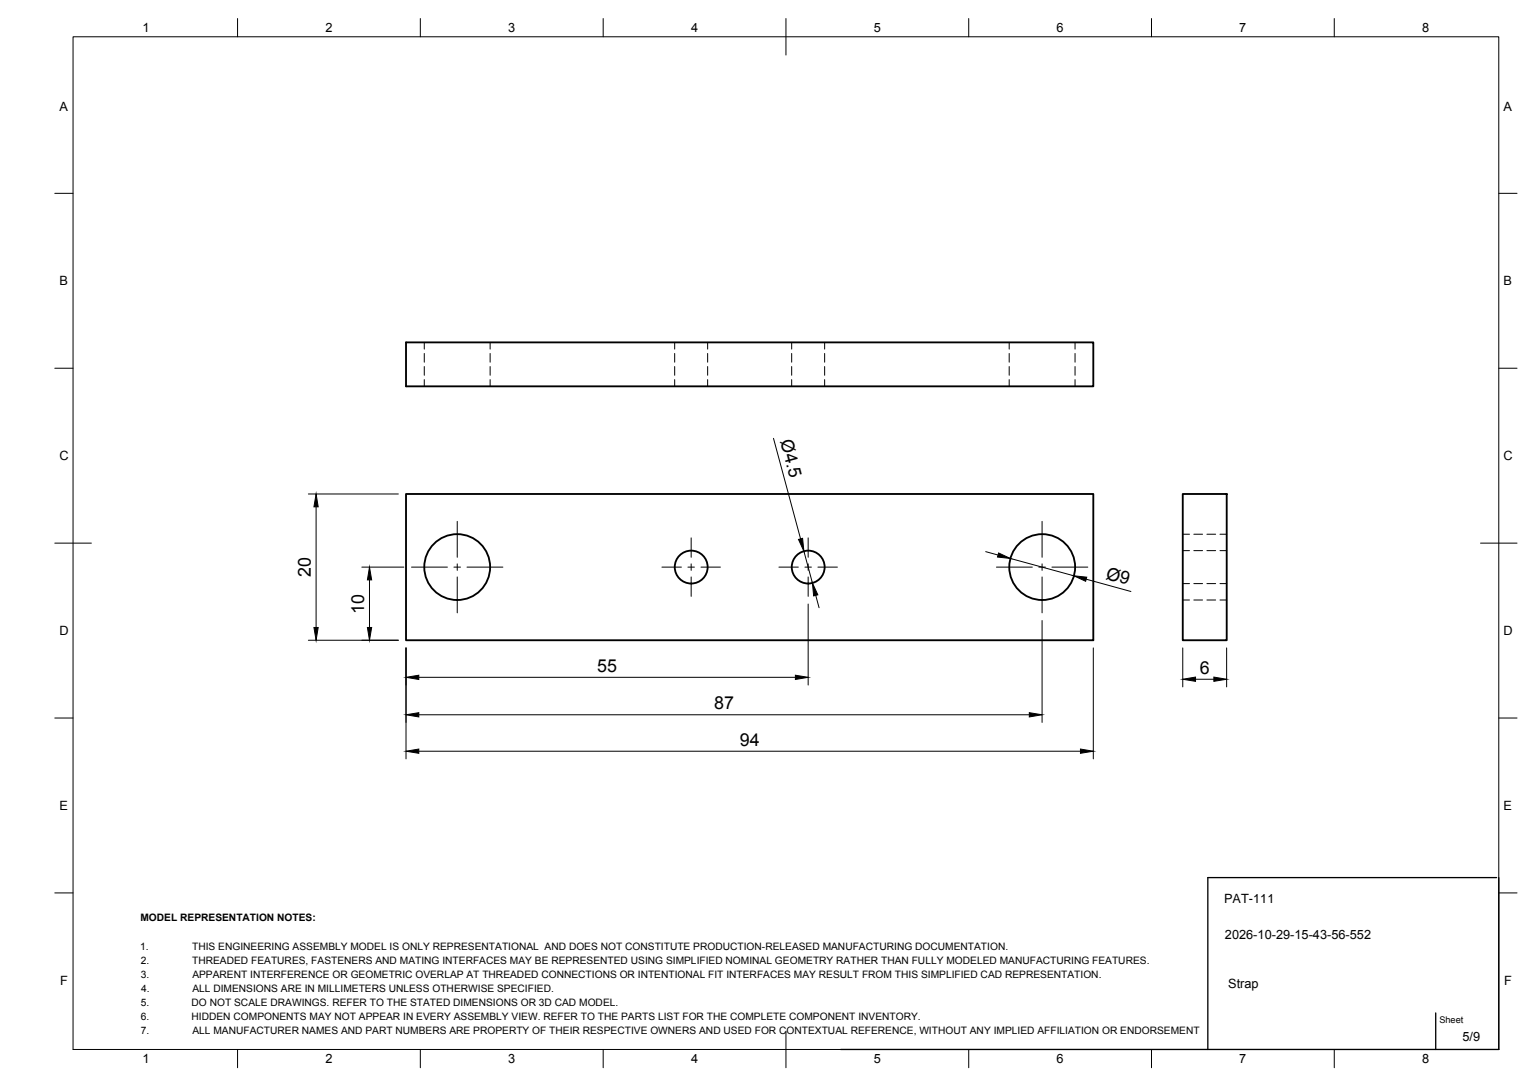
ISO-10303-21;
HEADER;
/* Generated by software containing ST-Developer
 * from STEP Tools, Inc. (www.steptools.com) 
 */

FILE_DESCRIPTION(
/* description */ ('Grid plate located blocks and clamp'),
/* implementation_level */ '2;1');

FILE_NAME(
/* name */ 'Strap.step',
/* time_stamp */ '2026-10-29T15:43:47-07:00',
/* author */ (''),
/* organization */ (''),
/* preprocessor_version */ 'ST-DEVELOPER v20.2',
/* originating_system */ 'Autodesk Translation Framework v15.17.0.0',
/* authorisation */ '');

FILE_SCHEMA (('AUTOMOTIVE_DESIGN { 1 0 10303 214 3 1 1 }'));
ENDSEC;

DATA;
#10=MECHANICAL_DESIGN_GEOMETRIC_PRESENTATION_REPRESENTATION('',(#172),#5702);
#146=SHAPE_REPRESENTATION_RELATIONSHIP('SRR','None',#5764,#158);
#158=ADVANCED_BREP_SHAPE_REPRESENTATION('',(#185),#5694);
#172=STYLED_ITEM('',(#5911),#185);
#185=MANIFOLD_SOLID_BREP('Body1',#3268);
#250=FACE_BOUND('',#811,.T.);
#251=FACE_BOUND('',#812,.T.);
#252=FACE_BOUND('',#813,.T.);
#253=FACE_BOUND('',#814,.T.);
#254=FACE_BOUND('',#816,.T.);
#255=FACE_BOUND('',#817,.T.);
#256=FACE_BOUND('',#818,.T.);
#257=FACE_BOUND('',#819,.T.);
#338=CIRCLE('',#3593,0.225);
#339=CIRCLE('',#3594,0.225);
#340=CIRCLE('',#3596,0.225);
#341=CIRCLE('',#3597,0.225);
#342=CIRCLE('',#3599,0.449999999999999);
#343=CIRCLE('',#3600,0.449999999999999);
#344=CIRCLE('',#3602,0.449999999999999);
#345=CIRCLE('',#3603,0.449999999999999);
#430=CYLINDRICAL_SURFACE('',#3592,0.225);
#431=CYLINDRICAL_SURFACE('',#3595,0.225);
#432=CYLINDRICAL_SURFACE('',#3598,0.449999999999999);
#433=CYLINDRICAL_SURFACE('',#3601,0.449999999999999);
#561=FACE_OUTER_BOUND('',#802,.T.);
#562=FACE_OUTER_BOUND('',#803,.T.);
#563=FACE_OUTER_BOUND('',#804,.T.);
#564=FACE_OUTER_BOUND('',#805,.T.);
#565=FACE_OUTER_BOUND('',#806,.T.);
#566=FACE_OUTER_BOUND('',#807,.T.);
#567=FACE_OUTER_BOUND('',#808,.T.);
#568=FACE_OUTER_BOUND('',#809,.T.);
#569=FACE_OUTER_BOUND('',#810,.T.);
#570=FACE_OUTER_BOUND('',#815,.T.);
#802=EDGE_LOOP('',(#2632,#2633,#2634,#2635));
#803=EDGE_LOOP('',(#2636,#2637,#2638,#2639));
#804=EDGE_LOOP('',(#2640,#2641,#2642,#2643));
#805=EDGE_LOOP('',(#2644,#2645,#2646,#2647));
#806=EDGE_LOOP('',(#2648,#2649,#2650,#2651));
#807=EDGE_LOOP('',(#2652,#2653,#2654,#2655));
#808=EDGE_LOOP('',(#2656,#2657,#2658,#2659));
#809=EDGE_LOOP('',(#2660,#2661,#2662,#2663));
#810=EDGE_LOOP('',(#2664,#2665,#2666,#2667));
#811=EDGE_LOOP('',(#2668));
#812=EDGE_LOOP('',(#2669));
#813=EDGE_LOOP('',(#2670));
#814=EDGE_LOOP('',(#2671));
#815=EDGE_LOOP('',(#2672,#2673,#2674,#2675));
#816=EDGE_LOOP('',(#2676));
#817=EDGE_LOOP('',(#2677));
#818=EDGE_LOOP('',(#2678));
#819=EDGE_LOOP('',(#2679));
#1077=LINE('',#5268,#1350);
#1078=LINE('',#5274,#1351);
#1079=LINE('',#5280,#1352);
#1080=LINE('',#5286,#1353);
#1081=LINE('',#5291,#1354);
#1082=LINE('',#5293,#1355);
#1083=LINE('',#5295,#1356);
#1084=LINE('',#5296,#1357);
#1085=LINE('',#5299,#1358);
#1086=LINE('',#5301,#1359);
#1087=LINE('',#5302,#1360);
#1088=LINE('',#5305,#1361);
#1089=LINE('',#5307,#1362);
#1090=LINE('',#5308,#1363);
#1091=LINE('',#5310,#1364);
#1092=LINE('',#5311,#1365);
#1350=VECTOR('',#4309,0.225);
#1351=VECTOR('',#4316,0.225);
#1352=VECTOR('',#4323,0.449999999999999);
#1353=VECTOR('',#4330,0.449999999999999);
#1354=VECTOR('',#4335,1.);
#1355=VECTOR('',#4336,1.);
#1356=VECTOR('',#4337,1.);
#1357=VECTOR('',#4338,1.);
#1358=VECTOR('',#4341,1.);
#1359=VECTOR('',#4342,1.);
#1360=VECTOR('',#4343,1.);
#1361=VECTOR('',#4346,1.);
#1362=VECTOR('',#4347,1.);
#1363=VECTOR('',#4348,1.);
#1364=VECTOR('',#4351,1.);
#1365=VECTOR('',#4352,1.);
#1607=VERTEX_POINT('',#5265);
#1608=VERTEX_POINT('',#5267);
#1609=VERTEX_POINT('',#5271);
#1610=VERTEX_POINT('',#5273);
#1611=VERTEX_POINT('',#5277);
#1612=VERTEX_POINT('',#5279);
#1613=VERTEX_POINT('',#5283);
#1614=VERTEX_POINT('',#5285);
#1615=VERTEX_POINT('',#5289);
#1616=VERTEX_POINT('',#5290);
#1617=VERTEX_POINT('',#5292);
#1618=VERTEX_POINT('',#5294);
#1619=VERTEX_POINT('',#5298);
#1620=VERTEX_POINT('',#5300);
#1621=VERTEX_POINT('',#5304);
#1622=VERTEX_POINT('',#5306);
#1966=EDGE_CURVE('',#1607,#1607,#338,.T.);
#1967=EDGE_CURVE('',#1607,#1608,#1077,.T.);
#1968=EDGE_CURVE('',#1608,#1608,#339,.T.);
#1969=EDGE_CURVE('',#1609,#1609,#340,.T.);
#1970=EDGE_CURVE('',#1609,#1610,#1078,.T.);
#1971=EDGE_CURVE('',#1610,#1610,#341,.T.);
#1972=EDGE_CURVE('',#1611,#1611,#342,.T.);
#1973=EDGE_CURVE('',#1611,#1612,#1079,.T.);
#1974=EDGE_CURVE('',#1612,#1612,#343,.T.);
#1975=EDGE_CURVE('',#1613,#1613,#344,.T.);
#1976=EDGE_CURVE('',#1613,#1614,#1080,.T.);
#1977=EDGE_CURVE('',#1614,#1614,#345,.T.);
#1978=EDGE_CURVE('',#1615,#1616,#1081,.T.);
#1979=EDGE_CURVE('',#1616,#1617,#1082,.T.);
#1980=EDGE_CURVE('',#1618,#1617,#1083,.T.);
#1981=EDGE_CURVE('',#1615,#1618,#1084,.T.);
#1982=EDGE_CURVE('',#1619,#1615,#1085,.T.);
#1983=EDGE_CURVE('',#1620,#1618,#1086,.T.);
#1984=EDGE_CURVE('',#1619,#1620,#1087,.T.);
#1985=EDGE_CURVE('',#1621,#1619,#1088,.T.);
#1986=EDGE_CURVE('',#1622,#1620,#1089,.T.);
#1987=EDGE_CURVE('',#1621,#1622,#1090,.T.);
#1988=EDGE_CURVE('',#1616,#1621,#1091,.T.);
#1989=EDGE_CURVE('',#1617,#1622,#1092,.T.);
#2632=ORIENTED_EDGE('',*,*,#1966,.F.);
#2633=ORIENTED_EDGE('',*,*,#1967,.T.);
#2634=ORIENTED_EDGE('',*,*,#1968,.F.);
#2635=ORIENTED_EDGE('',*,*,#1967,.F.);
#2636=ORIENTED_EDGE('',*,*,#1969,.F.);
#2637=ORIENTED_EDGE('',*,*,#1970,.T.);
#2638=ORIENTED_EDGE('',*,*,#1971,.F.);
#2639=ORIENTED_EDGE('',*,*,#1970,.F.);
#2640=ORIENTED_EDGE('',*,*,#1972,.F.);
#2641=ORIENTED_EDGE('',*,*,#1973,.T.);
#2642=ORIENTED_EDGE('',*,*,#1974,.F.);
#2643=ORIENTED_EDGE('',*,*,#1973,.F.);
#2644=ORIENTED_EDGE('',*,*,#1975,.F.);
#2645=ORIENTED_EDGE('',*,*,#1976,.T.);
#2646=ORIENTED_EDGE('',*,*,#1977,.F.);
#2647=ORIENTED_EDGE('',*,*,#1976,.F.);
#2648=ORIENTED_EDGE('',*,*,#1978,.T.);
#2649=ORIENTED_EDGE('',*,*,#1979,.T.);
#2650=ORIENTED_EDGE('',*,*,#1980,.F.);
#2651=ORIENTED_EDGE('',*,*,#1981,.F.);
#2652=ORIENTED_EDGE('',*,*,#1982,.T.);
#2653=ORIENTED_EDGE('',*,*,#1981,.T.);
#2654=ORIENTED_EDGE('',*,*,#1983,.F.);
#2655=ORIENTED_EDGE('',*,*,#1984,.F.);
#2656=ORIENTED_EDGE('',*,*,#1985,.T.);
#2657=ORIENTED_EDGE('',*,*,#1984,.T.);
#2658=ORIENTED_EDGE('',*,*,#1986,.F.);
#2659=ORIENTED_EDGE('',*,*,#1987,.F.);
#2660=ORIENTED_EDGE('',*,*,#1988,.T.);
#2661=ORIENTED_EDGE('',*,*,#1987,.T.);
#2662=ORIENTED_EDGE('',*,*,#1989,.F.);
#2663=ORIENTED_EDGE('',*,*,#1979,.F.);
#2664=ORIENTED_EDGE('',*,*,#1989,.T.);
#2665=ORIENTED_EDGE('',*,*,#1986,.T.);
#2666=ORIENTED_EDGE('',*,*,#1983,.T.);
#2667=ORIENTED_EDGE('',*,*,#1980,.T.);
#2668=ORIENTED_EDGE('',*,*,#1968,.T.);
#2669=ORIENTED_EDGE('',*,*,#1971,.T.);
#2670=ORIENTED_EDGE('',*,*,#1974,.T.);
#2671=ORIENTED_EDGE('',*,*,#1977,.T.);
#2672=ORIENTED_EDGE('',*,*,#1988,.F.);
#2673=ORIENTED_EDGE('',*,*,#1978,.F.);
#2674=ORIENTED_EDGE('',*,*,#1982,.F.);
#2675=ORIENTED_EDGE('',*,*,#1985,.F.);
#2676=ORIENTED_EDGE('',*,*,#1966,.T.);
#2677=ORIENTED_EDGE('',*,*,#1969,.T.);
#2678=ORIENTED_EDGE('',*,*,#1972,.T.);
#2679=ORIENTED_EDGE('',*,*,#1975,.T.);
#3031=PLANE('',#3604);
#3032=PLANE('',#3605);
#3033=PLANE('',#3606);
#3034=PLANE('',#3607);
#3035=PLANE('',#3608);
#3036=PLANE('',#3609);
#3182=ADVANCED_FACE('',(#561),#430,.F.);
#3183=ADVANCED_FACE('',(#562),#431,.F.);
#3184=ADVANCED_FACE('',(#563),#432,.F.);
#3185=ADVANCED_FACE('',(#564),#433,.F.);
#3186=ADVANCED_FACE('',(#565),#3031,.T.);
#3187=ADVANCED_FACE('',(#566),#3032,.T.);
#3188=ADVANCED_FACE('',(#567),#3033,.T.);
#3189=ADVANCED_FACE('',(#568),#3034,.T.);
#3190=ADVANCED_FACE('',(#569,#250,#251,#252,#253),#3035,.T.);
#3191=ADVANCED_FACE('',(#570,#254,#255,#256,#257),#3036,.F.);
#3268=CLOSED_SHELL('',(#3182,#3183,#3184,#3185,#3186,#3187,#3188,#3189,
#3190,#3191));
#3591=AXIS2_PLACEMENT_3D('',#5263,#4303,#4304);
#3592=AXIS2_PLACEMENT_3D('',#5264,#4305,#4306);
#3593=AXIS2_PLACEMENT_3D('',#5266,#4307,#4308);
#3594=AXIS2_PLACEMENT_3D('',#5269,#4310,#4311);
#3595=AXIS2_PLACEMENT_3D('',#5270,#4312,#4313);
#3596=AXIS2_PLACEMENT_3D('',#5272,#4314,#4315);
#3597=AXIS2_PLACEMENT_3D('',#5275,#4317,#4318);
#3598=AXIS2_PLACEMENT_3D('',#5276,#4319,#4320);
#3599=AXIS2_PLACEMENT_3D('',#5278,#4321,#4322);
#3600=AXIS2_PLACEMENT_3D('',#5281,#4324,#4325);
#3601=AXIS2_PLACEMENT_3D('',#5282,#4326,#4327);
#3602=AXIS2_PLACEMENT_3D('',#5284,#4328,#4329);
#3603=AXIS2_PLACEMENT_3D('',#5287,#4331,#4332);
#3604=AXIS2_PLACEMENT_3D('',#5288,#4333,#4334);
#3605=AXIS2_PLACEMENT_3D('',#5297,#4339,#4340);
#3606=AXIS2_PLACEMENT_3D('',#5303,#4344,#4345);
#3607=AXIS2_PLACEMENT_3D('',#5309,#4349,#4350);
#3608=AXIS2_PLACEMENT_3D('',#5312,#4353,#4354);
#3609=AXIS2_PLACEMENT_3D('',#5313,#4355,#4356);
#4303=DIRECTION('axis',(0.,0.,1.));
#4304=DIRECTION('refdir',(1.,0.,0.));
#4305=DIRECTION('center_axis',(0.,0.,1.));
#4306=DIRECTION('ref_axis',(1.,0.,0.));
#4307=DIRECTION('center_axis',(0.,0.,1.));
#4308=DIRECTION('ref_axis',(1.,0.,0.));
#4309=DIRECTION('',(0.,0.,1.));
#4310=DIRECTION('center_axis',(0.,0.,-1.));
#4311=DIRECTION('ref_axis',(1.,0.,0.));
#4312=DIRECTION('center_axis',(0.,0.,1.));
#4313=DIRECTION('ref_axis',(1.,0.,0.));
#4314=DIRECTION('center_axis',(0.,0.,1.));
#4315=DIRECTION('ref_axis',(1.,0.,0.));
#4316=DIRECTION('',(0.,0.,1.));
#4317=DIRECTION('center_axis',(0.,0.,-1.));
#4318=DIRECTION('ref_axis',(1.,0.,0.));
#4319=DIRECTION('center_axis',(0.,0.,1.));
#4320=DIRECTION('ref_axis',(1.,0.,0.));
#4321=DIRECTION('center_axis',(0.,0.,1.));
#4322=DIRECTION('ref_axis',(1.,0.,0.));
#4323=DIRECTION('',(0.,0.,1.));
#4324=DIRECTION('center_axis',(0.,0.,-1.));
#4325=DIRECTION('ref_axis',(1.,0.,0.));
#4326=DIRECTION('center_axis',(0.,0.,1.));
#4327=DIRECTION('ref_axis',(1.,0.,0.));
#4328=DIRECTION('center_axis',(0.,0.,1.));
#4329=DIRECTION('ref_axis',(1.,0.,0.));
#4330=DIRECTION('',(0.,0.,1.));
#4331=DIRECTION('center_axis',(0.,0.,-1.));
#4332=DIRECTION('ref_axis',(1.,0.,0.));
#4333=DIRECTION('center_axis',(0.,1.,0.));
#4334=DIRECTION('ref_axis',(-1.,0.,0.));
#4335=DIRECTION('',(-1.,0.,0.));
#4336=DIRECTION('',(0.,0.,1.));
#4337=DIRECTION('',(-1.,0.,0.));
#4338=DIRECTION('',(0.,0.,1.));
#4339=DIRECTION('center_axis',(1.,0.,0.));
#4340=DIRECTION('ref_axis',(0.,1.,0.));
#4341=DIRECTION('',(0.,1.,0.));
#4342=DIRECTION('',(0.,1.,0.));
#4343=DIRECTION('',(0.,0.,1.));
#4344=DIRECTION('center_axis',(0.,-1.,0.));
#4345=DIRECTION('ref_axis',(1.,0.,0.));
#4346=DIRECTION('',(1.,0.,0.));
#4347=DIRECTION('',(1.,0.,0.));
#4348=DIRECTION('',(0.,0.,1.));
#4349=DIRECTION('center_axis',(-1.,0.,0.));
#4350=DIRECTION('ref_axis',(0.,-1.,0.));
#4351=DIRECTION('',(0.,-1.,0.));
#4352=DIRECTION('',(0.,-1.,0.));
#4353=DIRECTION('center_axis',(0.,0.,1.));
#4354=DIRECTION('ref_axis',(1.,0.,0.));
#4355=DIRECTION('center_axis',(0.,0.,1.));
#4356=DIRECTION('ref_axis',(1.,0.,0.));
#5263=CARTESIAN_POINT('',(0.,0.,0.));
#5264=CARTESIAN_POINT('Origin',(10.,-0.8,6.42132034));
#5265=CARTESIAN_POINT('',(9.775,-0.8,6.52132034));
#5266=CARTESIAN_POINT('Origin',(10.,-0.8,6.52132034));
#5267=CARTESIAN_POINT('',(9.775,-0.8,7.12132034));
#5268=CARTESIAN_POINT('',(9.775,-0.8,6.42132034));
#5269=CARTESIAN_POINT('Origin',(10.,-0.8,7.12132034));
#5270=CARTESIAN_POINT('Origin',(10.,0.8,6.42132034));
#5271=CARTESIAN_POINT('',(9.775,0.8,6.52132034));
#5272=CARTESIAN_POINT('Origin',(10.,0.8,6.52132034));
#5273=CARTESIAN_POINT('',(9.775,0.8,7.12132034));
#5274=CARTESIAN_POINT('',(9.775,0.8,6.42132034));
#5275=CARTESIAN_POINT('Origin',(10.,0.8,7.12132034));
#5276=CARTESIAN_POINT('Origin',(10.,-4.,6.42132034));
#5277=CARTESIAN_POINT('',(9.55,-4.,6.52132034));
#5278=CARTESIAN_POINT('Origin',(10.,-4.,6.52132034));
#5279=CARTESIAN_POINT('',(9.55,-4.,7.12132034));
#5280=CARTESIAN_POINT('',(9.55,-4.,6.42132034));
#5281=CARTESIAN_POINT('Origin',(10.,-4.,7.12132034));
#5282=CARTESIAN_POINT('Origin',(10.,4.,6.42132034));
#5283=CARTESIAN_POINT('',(9.55,4.,6.52132034));
#5284=CARTESIAN_POINT('Origin',(10.,4.,6.52132034));
#5285=CARTESIAN_POINT('',(9.55,4.,7.12132034));
#5286=CARTESIAN_POINT('',(9.55,4.,6.42132034));
#5287=CARTESIAN_POINT('Origin',(10.,4.,7.12132034));
#5288=CARTESIAN_POINT('Origin',(11.,4.7,6.52132034));
#5289=CARTESIAN_POINT('',(11.,4.7,6.52132034));
#5290=CARTESIAN_POINT('',(9.,4.7,6.52132034));
#5291=CARTESIAN_POINT('',(11.,4.7,6.52132034));
#5292=CARTESIAN_POINT('',(9.,4.7,7.12132034));
#5293=CARTESIAN_POINT('',(9.,4.7,6.52132034));
#5294=CARTESIAN_POINT('',(11.,4.7,7.12132034));
#5295=CARTESIAN_POINT('',(11.,4.7,7.12132034));
#5296=CARTESIAN_POINT('',(11.,4.7,6.52132034));
#5297=CARTESIAN_POINT('Origin',(11.,-4.7,6.52132034));
#5298=CARTESIAN_POINT('',(11.,-4.7,6.52132034));
#5299=CARTESIAN_POINT('',(11.,-4.7,6.52132034));
#5300=CARTESIAN_POINT('',(11.,-4.7,7.12132034));
#5301=CARTESIAN_POINT('',(11.,-4.7,7.12132034));
#5302=CARTESIAN_POINT('',(11.,-4.7,6.52132034));
#5303=CARTESIAN_POINT('Origin',(9.,-4.7,6.52132034));
#5304=CARTESIAN_POINT('',(9.,-4.7,6.52132034));
#5305=CARTESIAN_POINT('',(9.,-4.7,6.52132034));
#5306=CARTESIAN_POINT('',(9.,-4.7,7.12132034));
#5307=CARTESIAN_POINT('',(9.,-4.7,7.12132034));
#5308=CARTESIAN_POINT('',(9.,-4.7,6.52132034));
#5309=CARTESIAN_POINT('Origin',(9.,4.7,6.52132034));
#5310=CARTESIAN_POINT('',(9.,4.7,6.52132034));
#5311=CARTESIAN_POINT('',(9.,4.7,7.12132034));
#5312=CARTESIAN_POINT('Origin',(10.,0.,7.12132034));
#5313=CARTESIAN_POINT('Origin',(10.,0.,6.52132034));
#5680=UNCERTAINTY_MEASURE_WITH_UNIT(LENGTH_MEASURE(0.001),#5703,
'DISTANCE_ACCURACY_VALUE',
'Maximum model space distance between geometric entities at asserted c
onnectivities');
#5688=UNCERTAINTY_MEASURE_WITH_UNIT(LENGTH_MEASURE(0.001),#5703,
'DISTANCE_ACCURACY_VALUE',
'Maximum model space distance between geometric entities at asserted c
onnectivities');
#5694=(
GEOMETRIC_REPRESENTATION_CONTEXT(3)
GLOBAL_UNCERTAINTY_ASSIGNED_CONTEXT((#5680))
GLOBAL_UNIT_ASSIGNED_CONTEXT((#5703,#5705,#5706))
REPRESENTATION_CONTEXT('','3D')
);
#5702=(
GEOMETRIC_REPRESENTATION_CONTEXT(3)
GLOBAL_UNCERTAINTY_ASSIGNED_CONTEXT((#5688))
GLOBAL_UNIT_ASSIGNED_CONTEXT((#5703,#5705,#5706))
REPRESENTATION_CONTEXT('','3D')
);
#5703=(
LENGTH_UNIT()
NAMED_UNIT(*)
SI_UNIT(.CENTI.,.METRE.)
);
#5705=(
NAMED_UNIT(*)
PLANE_ANGLE_UNIT()
SI_UNIT($,.RADIAN.)
);
#5706=(
NAMED_UNIT(*)
SI_UNIT($,.STERADIAN.)
SOLID_ANGLE_UNIT()
);
#5712=SHAPE_DEFINITION_REPRESENTATION(#5725,#5764);
#5725=PRODUCT_DEFINITION_SHAPE('',$,#5778);
#5764=SHAPE_REPRESENTATION('',(#3591),#5694);
#5772=PRODUCT_DEFINITION_CONTEXT('part definition',#5813,'design');
#5778=PRODUCT_DEFINITION('Strap','Strap',#5791,#5772);
#5791=PRODUCT_DEFINITION_FORMATION('',$,#5820);
#5813=APPLICATION_CONTEXT(
'Core Data for Automotive Mechanical Design Process');
#5814=PRODUCT_CONTEXT('part definition',#5813,'mechanical');
#5820=PRODUCT('Strap','Strap','Strap',(#5814));
#5905=COLOUR_RGB('Off White',0.89,0.88,0.83);
#5906=FILL_AREA_STYLE_COLOUR('',#5905);
#5907=FILL_AREA_STYLE('',(#5906));
#5908=SURFACE_STYLE_FILL_AREA(#5907);
#5909=SURFACE_SIDE_STYLE('',(#5908));
#5910=SURFACE_STYLE_USAGE(.BOTH.,#5909);
#5911=PRESENTATION_STYLE_ASSIGNMENT((#5910));
ENDSEC;
END-ISO-10303-21;
